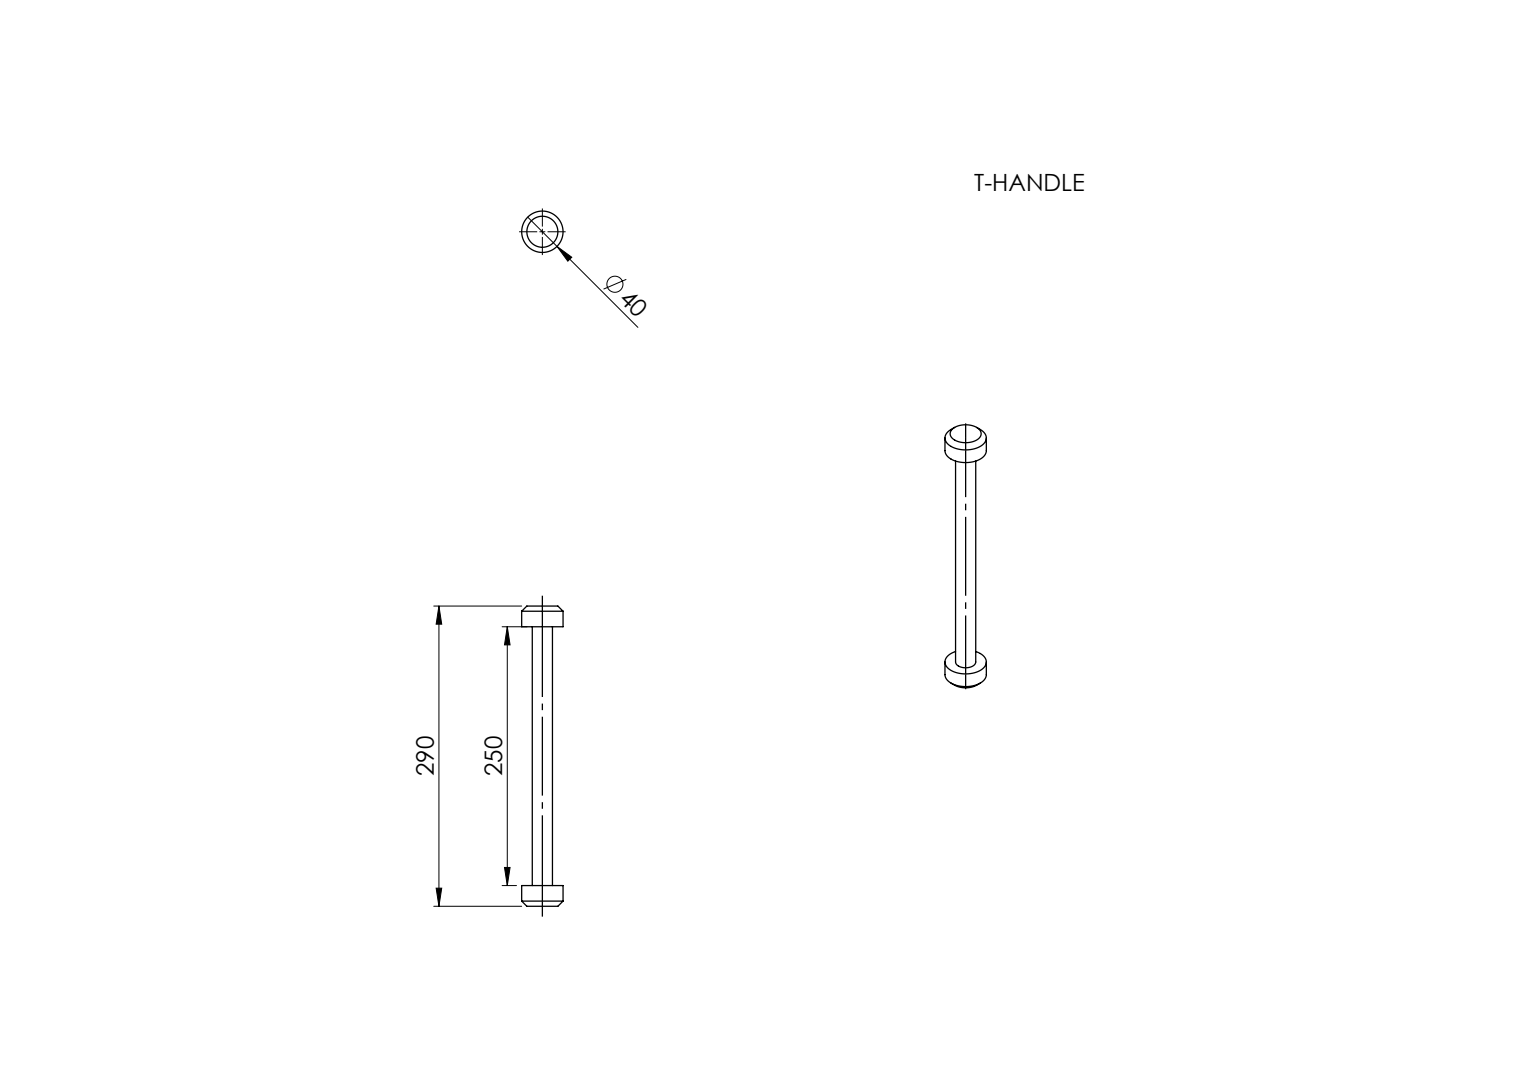
ISO-10303-21;
HEADER;
FILE_DESCRIPTION (('STEP AP203'),
    '1' );
FILE_NAME ('T-handle.step',
    '2026-09-28T05:57:06',
    ( '' ),
    ( '' ),
    'SwSTEP 2.0',
    'SolidWorks 2026',
    '' );
FILE_SCHEMA (( 'AUTOMOTIVE_DESIGN' ));
ENDSEC;

DATA;
#91=CARTESIAN_POINT ( 'NONE',  ( -1.040834085586084257E-14, -125.0000000000000000, 12.74999999999998934 ) ) ;
#177=LINE ( 'NONE', #29948, #5403 ) ;
#227=DIRECTION ( 'NONE',  ( 0.000000000000000000, -0.000000000000000000, 1.000000000000000000 ) ) ;
#268=ORIENTED_EDGE ( 'NONE', *, *, #28886, .F. ) ;
#419=VERTEX_POINT ( 'NONE', #17362 ) ;
#471=CARTESIAN_POINT ( 'NONE',  ( -1.040834085586084257E-14, -125.0000000000000000, 22.49999999999999289 ) ) ;
#473=ORIENTED_EDGE ( 'NONE', *, *, #25999, .F. ) ;
#566=CIRCLE ( 'NONE', #35714, 20.00000000000000000 ) ;
#851=MECHANICAL_CONTEXT ( 'NONE', #29772, 'mechanical' ) ;
#868=DIRECTION ( 'NONE',  ( 0.000000000000000000, 0.000000000000000000, -1.000000000000000000 ) ) ;
#1216=SHAPE_REPRESENTATION_RELATIONSHIP ( 'NONE' , 'NONE' ,  #40929, #17102 ) ;
#1231=DIRECTION ( 'NONE',  ( 0.000000000000000000, 0.000000000000000000, -1.000000000000000000 ) ) ;
#1234=CARTESIAN_POINT ( 'NONE',  ( -1.040834085586084257E-14, 145.0000000000000000, 22.49999999999999289 ) ) ;
#1383=LINE ( 'NONE', #34405, #18302 ) ;
#1425=DIRECTION ( 'NONE',  ( 0.000000000000000000, -1.000000000000000000, 0.000000000000000000 ) ) ;
#1545=LINE ( 'NONE', #40155, #18016 ) ;
#1660=CYLINDRICAL_SURFACE ( 'NONE', #36972, 20.00000000000000000 ) ;
#1786=CIRCLE ( 'NONE', #33508, 15.00000000000001066 ) ;
#1810=DIRECTION ( 'NONE',  ( 0.000000000000000000, 1.000000000000000000, 0.000000000000000000 ) ) ;
#1815=AXIS2_PLACEMENT_3D ( 'NONE', #36846, #20441, #33626 ) ;
#2067=CARTESIAN_POINT ( 'NONE',  ( -1.040834085586084257E-14, 139.9999999999999716, 2.499999999999992006 ) ) ;
#2073=ORIENTED_EDGE ( 'NONE', *, *, #14435, .F. ) ;
#2491=CARTESIAN_POINT ( 'NONE',  ( -1.040834085586084257E-14, 125.0000000000000000, 22.49999999999999289 ) ) ;
#3116=ORIENTED_EDGE ( 'NONE', *, *, #37024, .F. ) ;
#3335=VERTEX_POINT ( 'NONE', #22972 ) ;
#3448=EDGE_CURVE ( 'NONE', #21453, #419, #12086, .T. ) ;
#3451=CARTESIAN_POINT ( 'NONE',  ( -1.040834085586084257E-14, -145.0000000000000000, 22.49999999999999289 ) ) ;
#3477=DIRECTION ( 'NONE',  ( 0.000000000000000000, 0.000000000000000000, 1.000000000000000000 ) ) ;
#3738=LINE ( 'NONE', #6752, #8951 ) ;
#3889=CARTESIAN_POINT ( 'NONE',  ( -1.040834085586084257E-14, 145.0000000000000000, 22.49999999999999289 ) ) ;
#4161=ADVANCED_FACE ( 'NONE', ( #12961 ), #39308, .T. ) ;
#4188=DIRECTION ( 'NONE',  ( 0.000000000000000000, 1.000000000000000000, 0.000000000000000000 ) ) ;
#4342=VERTEX_POINT ( 'NONE', #5413 ) ;
#4391=FACE_OUTER_BOUND ( 'NONE', #42616, .T. ) ;
#4436=DIRECTION ( 'NONE',  ( 0.000000000000000000, 0.000000000000000000, 1.000000000000000000 ) ) ;
#4456=CYLINDRICAL_SURFACE ( 'NONE', #14879, 9.750000000000003553 ) ;
#4630=ORIENTED_EDGE ( 'NONE', *, *, #41333, .T. ) ;
#4816=EDGE_CURVE ( 'NONE', #28591, #27752, #8695, .T. ) ;
#4825=DIRECTION ( 'NONE',  ( -0.000000000000000000, -1.000000000000000000, -0.000000000000000000 ) ) ;
#4991=VECTOR ( 'NONE', #5574, 1000.000000000000000 ) ;
#5039=FACE_BOUND ( 'NONE', #22654, .T. ) ;
#5282=DIRECTION ( 'NONE',  ( 0.000000000000000000, 0.000000000000000000, 1.000000000000000000 ) ) ;
#5300=ORIENTED_EDGE ( 'NONE', *, *, #5846, .F. ) ;
#5341=ORIENTED_EDGE ( 'NONE', *, *, #32265, .F. ) ;
#5403=VECTOR ( 'NONE', #16964, 1000.000000000000000 ) ;
#5412=ADVANCED_FACE ( 'NONE', ( #20047 ), #40111, .T. ) ;
#5413=CARTESIAN_POINT ( 'NONE',  ( -1.040834085586084257E-14, -139.9999999999999716, 42.49999999999999289 ) ) ;
#5414=ADVANCED_FACE ( 'NONE', ( #13349, #26540 ), #39689, .F. ) ;
#5462=DIRECTION ( 'NONE',  ( 0.000000000000000000, 1.000000000000000000, 0.000000000000000000 ) ) ;
#5541=LINE ( 'NONE', #42409, #29579 ) ;
#5574=DIRECTION ( 'NONE',  ( -0.000000000000000000, 1.000000000000000000, -0.000000000000000000 ) ) ;
#5796=CARTESIAN_POINT ( 'NONE',  ( -1.040834085586084257E-14, 125.0000000000000000, 2.499999999999992006 ) ) ;
#5832=ORIENTED_EDGE ( 'NONE', *, *, #9357, .F. ) ;
#5846=EDGE_CURVE ( 'NONE', #39187, #5967, #12909, .T. ) ;
#5878=DIRECTION ( 'NONE',  ( 0.000000000000000000, 0.000000000000000000, -1.000000000000000000 ) ) ;
#5967=VERTEX_POINT ( 'NONE', #5796 ) ;
#6194=ORIENTED_EDGE ( 'NONE', *, *, #33703, .F. ) ;
#6272=DIRECTION ( 'NONE',  ( 0.000000000000000000, 0.000000000000000000, 1.000000000000000000 ) ) ;
#6295=AXIS2_PLACEMENT_3D ( 'NONE', #39092, #35241, #5878 ) ;
#6375=CARTESIAN_POINT ( 'NONE',  ( -8.571370657139810611E-15, -145.0000000000000000, 7.499999999999982236 ) ) ;
#6679=CARTESIAN_POINT ( 'NONE',  ( -8.265208957352971163E-15, -145.0000000000000000, 7.499999999999980460 ) ) ;
#6725=ORIENTED_EDGE ( 'NONE', *, *, #29092, .T. ) ;
#6752=CARTESIAN_POINT ( 'NONE',  ( -1.040834085586084257E-14, 125.0000000000000000, 12.74999999999998934 ) ) ;
#7066=CIRCLE ( 'NONE', #22933, 9.750000000000001776 ) ;
#7127=DIRECTION ( 'NONE',  ( -0.000000000000000000, -1.000000000000000000, -0.000000000000000000 ) ) ;
#7140=ORIENTED_EDGE ( 'NONE', *, *, #9357, .T. ) ;
#7254=FACE_OUTER_BOUND ( 'NONE', #12116, .T. ) ;
#7325=EDGE_CURVE ( 'NONE', #27752, #38572, #177, .T. ) ;
#7410=ORIENTED_EDGE ( 'NONE', *, *, #14435, .T. ) ;
#7450=AXIS2_PLACEMENT_3D ( 'NONE', #42023, #38585, #15478 ) ;
#7546=AXIS2_PLACEMENT_3D ( 'NONE', #35033, #5462, #15361 ) ;
#7648=DIRECTION ( 'NONE',  ( 0.000000000000000000, 0.000000000000000000, 1.000000000000000000 ) ) ;
#7735=AXIS2_PLACEMENT_3D ( 'NONE', #11600, #8398, #21548 ) ;
#7896=FACE_OUTER_BOUND ( 'NONE', #37238, .T. ) ;
#7974=FACE_OUTER_BOUND ( 'NONE', #12536, .T. ) ;
#8050=PRODUCT_DEFINITION_SHAPE ( 'NONE', 'NONE',  #24384 ) ;
#8094=ORIENTED_EDGE ( 'NONE', *, *, #32906, .F. ) ;
#8295=AXIS2_PLACEMENT_3D ( 'NONE', #20404, #1425, #41539 ) ;
#8353=FACE_OUTER_BOUND ( 'NONE', #19291, .T. ) ;
#8398=DIRECTION ( 'NONE',  ( 0.000000000000000000, -1.000000000000000000, 0.000000000000000000 ) ) ;
#8428=CYLINDRICAL_SURFACE ( 'NONE', #13259, 20.00000000000000355 ) ;
#8695=CIRCLE ( 'NONE', #1815, 14.99999999999998579 ) ;
#8706=ORIENTED_EDGE ( 'NONE', *, *, #5846, .T. ) ;
#8746=ORIENTED_EDGE ( 'NONE', *, *, #40574, .T. ) ;
#8807=ORIENTED_EDGE ( 'NONE', *, *, #31113, .T. ) ;
#8909=CARTESIAN_POINT ( 'NONE',  ( -7.959047257566134870E-15, 125.0000000000000000, 42.49999999999999289 ) ) ;
#8951=VECTOR ( 'NONE', #16868, 1000.000000000000000 ) ;
#9151=ORIENTED_EDGE ( 'NONE', *, *, #29092, .F. ) ;
#9230=CARTESIAN_POINT ( 'NONE',  ( -1.040834085586084257E-14, -139.9999999999999716, 22.49999999999999289 ) ) ;
#9234=DIRECTION ( 'NONE',  ( 0.000000000000000000, 0.000000000000000000, 1.000000000000000000 ) ) ;
#9270=ORIENTED_EDGE ( 'NONE', *, *, #18258, .F. ) ;
#9357=EDGE_CURVE ( 'NONE', #37654, #25583, #11643, .T. ) ;
#9744=CARTESIAN_POINT ( 'NONE',  ( -1.040834085586084257E-14, 145.0000000000000000, 22.49999999999999289 ) ) ;
#9794=CIRCLE ( 'NONE', #20826, 20.00000000000000355 ) ;
#10211=DIRECTION ( 'NONE',  ( 0.000000000000000000, 0.000000000000000000, -1.000000000000000000 ) ) ;
#10419=ORIENTED_EDGE ( 'NONE', *, *, #28886, .T. ) ;
#10429=UNCERTAINTY_MEASURE_WITH_UNIT (LENGTH_MEASURE( 1.000000000000000082E-05 ), #23882, 'distance_accuracy_value', 'NONE');
#10757=PRODUCT ( 'T-handle', 'T-handle', '', ( #851 ) ) ;
#10900=EDGE_CURVE ( 'NONE', #37654, #25373, #3738, .T. ) ;
#11112=DIRECTION ( 'NONE',  ( 0.000000000000000000, 0.000000000000000000, 1.000000000000000000 ) ) ;
#11370=ORIENTED_EDGE ( 'NONE', *, *, #37024, .T. ) ;
#11421=ORIENTED_EDGE ( 'NONE', *, *, #18258, .T. ) ;
#11600=CARTESIAN_POINT ( 'NONE',  ( -1.040834085586084257E-14, -145.0000000000000000, 22.49999999999999289 ) ) ;
#11643=CIRCLE ( 'NONE', #23396, 9.750000000000001776 ) ;
#12039=DIRECTION ( 'NONE',  ( 0.000000000000000000, 1.000000000000000000, 0.000000000000000000 ) ) ;
#12086=CIRCLE ( 'NONE', #29349, 15.00000000000001066 ) ;
#12116=EDGE_LOOP ( 'NONE', ( #15883, #7410, #35250, #37009 ) ) ;
#12183=EDGE_LOOP ( 'NONE', ( #16198, #17481, #11421, #28012 ) ) ;
#12520=DIRECTION ( 'NONE',  ( 0.000000000000000000, 0.000000000000000000, 1.000000000000000000 ) ) ;
#12536=EDGE_LOOP ( 'NONE', ( #2073, #42065, #22291, #32171 ) ) ;
#12645=CARTESIAN_POINT ( 'NONE',  ( -1.040834085586084257E-14, -145.0000000000000000, 42.49999999999999289 ) ) ;
#12873=CYLINDRICAL_SURFACE ( 'NONE', #7450, 9.750000000000003553 ) ;
#12909=CIRCLE ( 'NONE', #19152, 20.00000000000000355 ) ;
#12961=FACE_OUTER_BOUND ( 'NONE', #15238, .T. ) ;
#13031=LINE ( 'NONE', #6375, #28845 ) ;
#13034=AXIS2_PLACEMENT_3D ( 'NONE', #24309, #31209, #4436 ) ;
#13165=ORIENTED_EDGE ( 'NONE', *, *, #32906, .T. ) ;
#13259=AXIS2_PLACEMENT_3D ( 'NONE', #30871, #21581, #20715 ) ;
#13286=ORIENTED_EDGE ( 'NONE', *, *, #35143, .F. ) ;
#13349=FACE_BOUND ( 'NONE', #14661, .T. ) ;
#13398=EDGE_CURVE ( 'NONE', #27752, #28591, #24497, .T. ) ;
#13583=VERTEX_POINT ( 'NONE', #14542 ) ;
#13757=ADVANCED_FACE ( 'NONE', ( #5039, #4391 ), #18184, .F. ) ;
#13859=CIRCLE ( 'NONE', #6295, 20.00000000000000000 ) ;
#14121=( NAMED_UNIT ( * ) PLANE_ANGLE_UNIT ( ) SI_UNIT ( $, .RADIAN. ) );
#14435=EDGE_CURVE ( 'NONE', #28591, #34451, #1545, .T. ) ;
#14505=DIRECTION ( 'NONE',  ( 0.000000000000000000, -0.000000000000000000, 1.000000000000000000 ) ) ;
#14542=CARTESIAN_POINT ( 'NONE',  ( -9.214310226692173294E-15, -125.0000000000000000, 32.24999999999999289 ) ) ;
#14620=ORIENTED_EDGE ( 'NONE', *, *, #16955, .T. ) ;
#14661=EDGE_LOOP ( 'NONE', ( #6194, #9270 ) ) ;
#14780=ORIENTED_EDGE ( 'NONE', *, *, #27800, .F. ) ;
#14792=DIRECTION ( 'NONE',  ( -0.000000000000000000, -1.000000000000000000, -0.000000000000000000 ) ) ;
#14879=AXIS2_PLACEMENT_3D ( 'NONE', #21281, #30796, #1231 ) ;
#15101=DIRECTION ( 'NONE',  ( 0.000000000000000000, -1.000000000000000000, 0.000000000000000000 ) ) ;
#15238=EDGE_LOOP ( 'NONE', ( #15424, #36816, #11370, #14620 ) ) ;
#15361=DIRECTION ( 'NONE',  ( 0.000000000000000000, 0.000000000000000000, -1.000000000000000000 ) ) ;
#15424=ORIENTED_EDGE ( 'NONE', *, *, #19650, .F. ) ;
#15442=ORIENTED_EDGE ( 'NONE', *, *, #39183, .F. ) ;
#15478=DIRECTION ( 'NONE',  ( 0.000000000000000000, 0.000000000000000000, -1.000000000000000000 ) ) ;
#15625=ORIENTED_EDGE ( 'NONE', *, *, #31113, .F. ) ;
#15877=DIRECTION ( 'NONE',  ( 0.000000000000000000, -1.000000000000000000, 0.000000000000000000 ) ) ;
#15883=ORIENTED_EDGE ( 'NONE', *, *, #4816, .F. ) ;
#16198=ORIENTED_EDGE ( 'NONE', *, *, #40574, .F. ) ;
#16519=CIRCLE ( 'NONE', #30358, 9.750000000000001776 ) ;
#16610=AXIS2_PLACEMENT_3D ( 'NONE', #24461, #17732, #25103 ) ;
#16868=DIRECTION ( 'NONE',  ( -0.000000000000000000, -1.000000000000000000, -0.000000000000000000 ) ) ;
#16900=AXIS2_PLACEMENT_3D ( 'NONE', #9744, #22925, #17266 ) ;
#16955=EDGE_CURVE ( 'NONE', #5967, #39187, #9794, .T. ) ;
#16964=DIRECTION ( 'NONE',  ( 0.000000000000000000, -0.7071067811865487940, -0.7071067811865463515 ) ) ;
#17102=ADVANCED_BREP_SHAPE_REPRESENTATION ( '', ( #29300, #39998 ), #28294 ) ;
#17266=DIRECTION ( 'NONE',  ( 0.000000000000000000, 0.000000000000000000, -1.000000000000000000 ) ) ;
#17333=CARTESIAN_POINT ( 'NONE',  ( -1.040834085586084257E-14, -145.0000000000000000, 22.49999999999999289 ) ) ;
#17362=CARTESIAN_POINT ( 'NONE',  ( -1.040834085586084257E-14, -145.0000000000000000, 37.50000000000000711 ) ) ;
#17481=ORIENTED_EDGE ( 'NONE', *, *, #35143, .T. ) ;
#17732=DIRECTION ( 'NONE',  ( 0.000000000000000000, -1.000000000000000000, 0.000000000000000000 ) ) ;
#17992=DIRECTION ( 'NONE',  ( 0.000000000000000000, 0.000000000000000000, 1.000000000000000000 ) ) ;
#18016=VECTOR ( 'NONE', #30678, 1000.000000000000000 ) ;
#18184=PLANE ( 'NONE',  #29981 ) ;
#18258=EDGE_CURVE ( 'NONE', #13583, #25373, #7066, .T. ) ;
#18302=VECTOR ( 'NONE', #4825, 1000.000000000000000 ) ;
#18510=CONICAL_SURFACE ( 'NONE', #23327, 15.00000000000001421, 0.7853981633974469467 ) ;
#18565=ADVANCED_FACE ( 'NONE', ( #37984 ), #8428, .T. ) ;
#18586=CARTESIAN_POINT ( 'NONE',  ( -1.040834085586084257E-14, 125.0000000000000000, 22.49999999999999289 ) ) ;
#18658=DIRECTION ( 'NONE',  ( 0.000000000000000000, 1.000000000000000000, 0.000000000000000000 ) ) ;
#18945=FACE_OUTER_BOUND ( 'NONE', #33907, .T. ) ;
#19152=AXIS2_PLACEMENT_3D ( 'NONE', #32135, #12039, #9234 ) ;
#19291=EDGE_LOOP ( 'NONE', ( #4630, #39311, #8706, #3116 ) ) ;
#19323=EDGE_LOOP ( 'NONE', ( #8807, #6725, #10419, #14780 ) ) ;
#19345=CARTESIAN_POINT ( 'NONE',  ( -1.040834085586084257E-14, 145.0000000000000000, 7.500000000000003553 ) ) ;
#19362=CARTESIAN_POINT ( 'NONE',  ( -7.959047257566134870E-15, -145.0000000000000000, 2.499999999999992006 ) ) ;
#19418=DIRECTION ( 'NONE',  ( 0.000000000000000000, 1.000000000000000000, 0.000000000000000000 ) ) ;
#19650=EDGE_CURVE ( 'NONE', #34451, #39187, #1383, .T. ) ;
#19715=CARTESIAN_POINT ( 'NONE',  ( -1.040834085586084257E-14, -145.0000000000000000, 22.49999999999999289 ) ) ;
#19834=CARTESIAN_POINT ( 'NONE',  ( -1.040834085586084257E-14, 145.0000000000000000, 22.49999999999999289 ) ) ;
#19857=AXIS2_PLACEMENT_3D ( 'NONE', #20371, #30962, #7648 ) ;
#19982=CONICAL_SURFACE ( 'NONE', #8295, 14.99999999999998579, 0.7853981633974466137 ) ;
#20047=FACE_OUTER_BOUND ( 'NONE', #35756, .T. ) ;
#20371=CARTESIAN_POINT ( 'NONE',  ( -1.040834085586084257E-14, -125.0000000000000000, 22.49999999999999289 ) ) ;
#20404=CARTESIAN_POINT ( 'NONE',  ( -1.040834085586084257E-14, 145.0000000000000000, 22.49999999999999289 ) ) ;
#20441=DIRECTION ( 'NONE',  ( 0.000000000000000000, 1.000000000000000000, 0.000000000000000000 ) ) ;
#20539=CARTESIAN_POINT ( 'NONE',  ( -7.959047257566134870E-15, 139.9999999999999716, 42.49999999999999289 ) ) ;
#20576=DIRECTION ( 'NONE',  ( 0.000000000000000000, 0.000000000000000000, 1.000000000000000000 ) ) ;
#20624=CIRCLE ( 'NONE', #7546, 20.00000000000000000 ) ;
#20715=DIRECTION ( 'NONE',  ( 0.000000000000000000, 0.000000000000000000, 1.000000000000000000 ) ) ;
#20793=FACE_OUTER_BOUND ( 'NONE', #25894, .T. ) ;
#20826=AXIS2_PLACEMENT_3D ( 'NONE', #37652, #21456, #17992 ) ;
#20837=ORIENTED_EDGE ( 'NONE', *, *, #33703, .T. ) ;
#20943=EDGE_CURVE ( 'NONE', #419, #21453, #1786, .T. ) ;
#21048=( NAMED_UNIT ( * ) SI_UNIT ( $, .STERADIAN. ) SOLID_ANGLE_UNIT ( ) );
#21110=PLANE ( 'NONE',  #7735 ) ;
#21281=CARTESIAN_POINT ( 'NONE',  ( -1.040834085586084257E-14, 125.0000000000000000, 22.49999999999999289 ) ) ;
#21453=VERTEX_POINT ( 'NONE', #6679 ) ;
#21456=DIRECTION ( 'NONE',  ( 0.000000000000000000, 1.000000000000000000, 0.000000000000000000 ) ) ;
#21498=CONICAL_SURFACE ( 'NONE', #40096, 15.00000000000001421, 0.7853981633974469467 ) ;
#21548=DIRECTION ( 'NONE',  ( 0.000000000000000000, -0.000000000000000000, -1.000000000000000000 ) ) ;
#21581=DIRECTION ( 'NONE',  ( -0.000000000000000000, 1.000000000000000000, -0.000000000000000000 ) ) ;
#21733=CONICAL_SURFACE ( 'NONE', #36204, 14.99999999999998579, 0.7853981633974466137 ) ;
#22009=ADVANCED_FACE ( 'NONE', ( #27338 ), #4456, .T. ) ;
#22291=ORIENTED_EDGE ( 'NONE', *, *, #7325, .T. ) ;
#22512=ADVANCED_FACE ( 'NONE', ( #8353 ), #1660, .T. ) ;
#22513=CARTESIAN_POINT ( 'NONE',  ( -1.040834085586084257E-14, -145.0000000000000000, 37.50000000000000711 ) ) ;
#22594=LINE ( 'NONE', #12645, #28388 ) ;
#22608=DIRECTION ( 'NONE',  ( 0.000000000000000000, -1.000000000000000000, 0.000000000000000000 ) ) ;
#22654=EDGE_LOOP ( 'NONE', ( #7140, #8746 ) ) ;
#22925=DIRECTION ( 'NONE',  ( -0.000000000000000000, -1.000000000000000000, -0.000000000000000000 ) ) ;
#22933=AXIS2_PLACEMENT_3D ( 'NONE', #471, #26983, #3477 ) ;
#22972=CARTESIAN_POINT ( 'NONE',  ( -7.959047257566134870E-15, -125.0000000000000000, 2.499999999999992006 ) ) ;
#23303=CARTESIAN_POINT ( 'NONE',  ( -1.040834085586084257E-14, -125.0000000000000000, 22.49999999999999289 ) ) ;
#23327=AXIS2_PLACEMENT_3D ( 'NONE', #17333, #4188, #20576 ) ;
#23396=AXIS2_PLACEMENT_3D ( 'NONE', #18586, #28532, #12520 ) ;
#23614=ADVANCED_FACE ( 'NONE', ( #7974 ), #21733, .T. ) ;
#23882=( LENGTH_UNIT ( ) NAMED_UNIT ( * ) SI_UNIT ( .MILLI., .METRE. ) );
#24309=CARTESIAN_POINT ( 'NONE',  ( -1.040834085586084257E-14, -145.0000000000000000, 22.49999999999999289 ) ) ;
#24384=PRODUCT_DEFINITION ( 'UNKNOWN', '', #28392, #39072 ) ;
#24461=CARTESIAN_POINT ( 'NONE',  ( -1.040834085586084257E-14, 139.9999999999999716, 22.49999999999999289 ) ) ;
#24470=AXIS2_PLACEMENT_3D ( 'NONE', #31409, #34860, #5282 ) ;
#24497=CIRCLE ( 'NONE', #24470, 14.99999999999998579 ) ;
#24743=CARTESIAN_POINT ( 'NONE',  ( 0.000000000000000000, 0.000000000000000000, 0.000000000000000000 ) ) ;
#25103=DIRECTION ( 'NONE',  ( 0.000000000000000000, 0.000000000000000000, 1.000000000000000000 ) ) ;
#25167=ORIENTED_EDGE ( 'NONE', *, *, #4816, .T. ) ;
#25227=CARTESIAN_POINT ( 'NONE',  ( -1.040834085586084257E-14, -125.0000000000000000, 22.49999999999999289 ) ) ;
#25373=VERTEX_POINT ( 'NONE', #91 ) ;
#25583=VERTEX_POINT ( 'NONE', #27471 ) ;
#25843=EDGE_CURVE ( 'NONE', #34451, #38572, #34575, .T. ) ;
#25894=EDGE_LOOP ( 'NONE', ( #32902, #28883, #15625, #8094 ) ) ;
#25999=EDGE_CURVE ( 'NONE', #32995, #3335, #13859, .T. ) ;
#26540=FACE_OUTER_BOUND ( 'NONE', #32275, .T. ) ;
#26766=LINE ( 'NONE', #39919, #30255 ) ;
#26956=DIRECTION ( 'NONE',  ( 0.000000000000000000, 1.000000000000000000, 0.000000000000000000 ) ) ;
#26983=DIRECTION ( 'NONE',  ( 0.000000000000000000, 1.000000000000000000, 0.000000000000000000 ) ) ;
#26991=ADVANCED_FACE ( 'NONE', ( #29569 ), #21498, .T. ) ;
#27338=FACE_OUTER_BOUND ( 'NONE', #12183, .T. ) ;
#27471=CARTESIAN_POINT ( 'NONE',  ( -9.214310226692173294E-15, 125.0000000000000000, 32.24999999999999289 ) ) ;
#27752=VERTEX_POINT ( 'NONE', #19345 ) ;
#27800=EDGE_CURVE ( 'NONE', #4342, #32995, #22594, .T. ) ;
#27987=DIRECTION ( 'NONE',  ( 0.000000000000000000, 0.000000000000000000, -1.000000000000000000 ) ) ;
#28012=ORIENTED_EDGE ( 'NONE', *, *, #10900, .F. ) ;
#28294=( GEOMETRIC_REPRESENTATION_CONTEXT ( 3 ) GLOBAL_UNCERTAINTY_ASSIGNED_CONTEXT ( ( #10429 ) ) GLOBAL_UNIT_ASSIGNED_CONTEXT ( ( #23882, #14121, #21048 ) ) REPRESENTATION_CONTEXT ( 'NONE', 'WORKASPACE' ) );
#28388=VECTOR ( 'NONE', #38993, 1000.000000000000000 ) ;
#28392=PRODUCT_DEFINITION_FORMATION_WITH_SPECIFIED_SOURCE ( 'ANY', '', #10757, .NOT_KNOWN. ) ;
#28403=ORIENTED_EDGE ( 'NONE', *, *, #39183, .T. ) ;
#28532=DIRECTION ( 'NONE',  ( 0.000000000000000000, 1.000000000000000000, 0.000000000000000000 ) ) ;
#28591=VERTEX_POINT ( 'NONE', #40945 ) ;
#28677=DIRECTION ( 'NONE',  ( 0.000000000000000000, 0.000000000000000000, -1.000000000000000000 ) ) ;
#28755=ADVANCED_FACE ( 'NONE', ( #37952 ), #21110, .T. ) ;
#28790=LINE ( 'NONE', #22513, #34355 ) ;
#28845=VECTOR ( 'NONE', #39167, 1000.000000000000000 ) ;
#28883=ORIENTED_EDGE ( 'NONE', *, *, #32265, .T. ) ;
#28886=EDGE_CURVE ( 'NONE', #3335, #32995, #29793, .T. ) ;
#29092=EDGE_CURVE ( 'NONE', #32177, #3335, #42233, .T. ) ;
#29290=ORIENTED_EDGE ( 'NONE', *, *, #13398, .T. ) ;
#29300=MANIFOLD_SOLID_BREP ( 'Chamfer1', #41117 ) ;
#29349=AXIS2_PLACEMENT_3D ( 'NONE', #19715, #29873, #10211 ) ;
#29569=FACE_OUTER_BOUND ( 'NONE', #33567, .T. ) ;
#29579=VECTOR ( 'NONE', #36159, 1000.000000000000000 ) ;
#29772=APPLICATION_CONTEXT ( 'configuration controlled 3d designs of mechanical parts and assemblies' ) ;
#29793=CIRCLE ( 'NONE', #39423, 20.00000000000000000 ) ;
#29873=DIRECTION ( 'NONE',  ( 0.000000000000000000, -1.000000000000000000, 0.000000000000000000 ) ) ;
#29948=CARTESIAN_POINT ( 'NONE',  ( -1.040834085586084257E-14, 145.0000000000000000, 7.500000000000007105 ) ) ;
#29981=AXIS2_PLACEMENT_3D ( 'NONE', #31376, #1810, #14505 ) ;
#30058=CARTESIAN_POINT ( 'NONE',  ( -1.040834085586084257E-14, -125.0000000000000000, 42.49999999999999289 ) ) ;
#30255=VECTOR ( 'NONE', #7127, 1000.000000000000000 ) ;
#30358=AXIS2_PLACEMENT_3D ( 'NONE', #2491, #18658, #41742 ) ;
#30437=DIRECTION ( 'NONE',  ( 0.000000000000000000, -1.000000000000000000, 0.000000000000000000 ) ) ;
#30678=DIRECTION ( 'NONE',  ( 8.659560562354918067E-17, -0.7071067811865487940, 0.7071067811865463515 ) ) ;
#30796=DIRECTION ( 'NONE',  ( -0.000000000000000000, -1.000000000000000000, -0.000000000000000000 ) ) ;
#30871=CARTESIAN_POINT ( 'NONE',  ( -1.040834085586084257E-14, -145.0000000000000000, 22.49999999999999289 ) ) ;
#30933=ORIENTED_EDGE ( 'NONE', *, *, #20943, .F. ) ;
#30962=DIRECTION ( 'NONE',  ( 0.000000000000000000, 1.000000000000000000, 0.000000000000000000 ) ) ;
#31106=ORIENTED_EDGE ( 'NONE', *, *, #10900, .T. ) ;
#31113=EDGE_CURVE ( 'NONE', #4342, #32177, #566, .T. ) ;
#31209=DIRECTION ( 'NONE',  ( -0.000000000000000000, 1.000000000000000000, -0.000000000000000000 ) ) ;
#31262=ADVANCED_FACE ( 'NONE', ( #18945 ), #12873, .T. ) ;
#31376=CARTESIAN_POINT ( 'NONE',  ( -1.040834085586084257E-14, 125.0000000000000000, 22.49999999999999289 ) ) ;
#31386=DIRECTION ( 'NONE',  ( 0.000000000000000000, 0.7071067811865484609, 0.7071067811865465735 ) ) ;
#31409=CARTESIAN_POINT ( 'NONE',  ( -1.040834085586084257E-14, 145.0000000000000000, 22.49999999999999289 ) ) ;
#31544=CARTESIAN_POINT ( 'NONE',  ( -1.040834085586084257E-14, -145.0000000000000000, 22.49999999999999289 ) ) ;
#32135=CARTESIAN_POINT ( 'NONE',  ( -1.040834085586084257E-14, 125.0000000000000000, 22.49999999999999289 ) ) ;
#32171=ORIENTED_EDGE ( 'NONE', *, *, #25843, .F. ) ;
#32177=VERTEX_POINT ( 'NONE', #32499 ) ;
#32265=EDGE_CURVE ( 'NONE', #21453, #32177, #13031, .T. ) ;
#32275=EDGE_LOOP ( 'NONE', ( #473, #268 ) ) ;
#32499=CARTESIAN_POINT ( 'NONE',  ( -7.959047257566134870E-15, -139.9999999999999716, 2.499999999999992006 ) ) ;
#32505=ADVANCED_FACE ( 'NONE', ( #20793 ), #18510, .T. ) ;
#32902=ORIENTED_EDGE ( 'NONE', *, *, #3448, .F. ) ;
#32906=EDGE_CURVE ( 'NONE', #419, #4342, #28790, .T. ) ;
#32995=VERTEX_POINT ( 'NONE', #30058 ) ;
#33242=DIRECTION ( 'NONE',  ( 0.000000000000000000, -0.000000000000000000, -1.000000000000000000 ) ) ;
#33508=AXIS2_PLACEMENT_3D ( 'NONE', #31544, #15101, #40787 ) ;
#33544=EDGE_LOOP ( 'NONE', ( #40730, #40717 ) ) ;
#33567=EDGE_LOOP ( 'NONE', ( #5341, #30933, #13165, #15442 ) ) ;
#33626=DIRECTION ( 'NONE',  ( 0.000000000000000000, 0.000000000000000000, 1.000000000000000000 ) ) ;
#33703=EDGE_CURVE ( 'NONE', #25373, #13583, #35040, .T. ) ;
#33804=AXIS2_PLACEMENT_3D ( 'NONE', #42427, #15877, #38991 ) ;
#33907=EDGE_LOOP ( 'NONE', ( #13286, #5832, #31106, #20837 ) ) ;
#34355=VECTOR ( 'NONE', #31386, 1000.000000000000000 ) ;
#34405=CARTESIAN_POINT ( 'NONE',  ( -7.959047257566134870E-15, 145.0000000000000000, 42.49999999999999289 ) ) ;
#34451=VERTEX_POINT ( 'NONE', #20539 ) ;
#34575=CIRCLE ( 'NONE', #16610, 20.00000000000000355 ) ;
#34665=CARTESIAN_POINT ( 'NONE',  ( -1.040834085586084257E-14, 125.0000000000000000, 12.74999999999998934 ) ) ;
#34725=SHAPE_DEFINITION_REPRESENTATION ( #8050, #40929 ) ;
#34860=DIRECTION ( 'NONE',  ( 0.000000000000000000, 1.000000000000000000, 0.000000000000000000 ) ) ;
#35033=CARTESIAN_POINT ( 'NONE',  ( -1.040834085586084257E-14, -139.9999999999999716, 22.49999999999999289 ) ) ;
#35040=CIRCLE ( 'NONE', #19857, 9.750000000000001776 ) ;
#35143=EDGE_CURVE ( 'NONE', #25583, #13583, #26766, .T. ) ;
#35241=DIRECTION ( 'NONE',  ( 0.000000000000000000, -1.000000000000000000, 0.000000000000000000 ) ) ;
#35250=ORIENTED_EDGE ( 'NONE', *, *, #41333, .F. ) ;
#35714=AXIS2_PLACEMENT_3D ( 'NONE', #9230, #41603, #38377 ) ;
#35756=EDGE_LOOP ( 'NONE', ( #29290, #25167 ) ) ;
#36159=DIRECTION ( 'NONE',  ( -0.000000000000000000, -1.000000000000000000, -0.000000000000000000 ) ) ;
#36204=AXIS2_PLACEMENT_3D ( 'NONE', #3889, #30437, #868 ) ;
#36285=ORIENTED_EDGE ( 'NONE', *, *, #16955, .F. ) ;
#36816=ORIENTED_EDGE ( 'NONE', *, *, #25843, .T. ) ;
#36846=CARTESIAN_POINT ( 'NONE',  ( -1.040834085586084257E-14, 145.0000000000000000, 22.49999999999999289 ) ) ;
#36972=AXIS2_PLACEMENT_3D ( 'NONE', #1234, #14792, #27987 ) ;
#37009=ORIENTED_EDGE ( 'NONE', *, *, #7325, .F. ) ;
#37024=EDGE_CURVE ( 'NONE', #38572, #5967, #5541, .T. ) ;
#37238=EDGE_LOOP ( 'NONE', ( #9151, #28403, #40355, #42120 ) ) ;
#37629=AXIS2_PLACEMENT_3D ( 'NONE', #23303, #39269, #33242 ) ;
#37652=CARTESIAN_POINT ( 'NONE',  ( -1.040834085586084257E-14, 125.0000000000000000, 22.49999999999999289 ) ) ;
#37654=VERTEX_POINT ( 'NONE', #34665 ) ;
#37889=DIRECTION ( 'NONE',  ( 1.000000000000000000, 0.000000000000000000, 0.000000000000000000 ) ) ;
#37952=FACE_OUTER_BOUND ( 'NONE', #33544, .T. ) ;
#37984=FACE_OUTER_BOUND ( 'NONE', #19323, .T. ) ;
#38345=ADVANCED_FACE ( 'NONE', ( #7896 ), #41311, .T. ) ;
#38377=DIRECTION ( 'NONE',  ( 0.000000000000000000, 0.000000000000000000, -1.000000000000000000 ) ) ;
#38572=VERTEX_POINT ( 'NONE', #2067 ) ;
#38585=DIRECTION ( 'NONE',  ( -0.000000000000000000, -1.000000000000000000, -0.000000000000000000 ) ) ;
#38635=CIRCLE ( 'NONE', #33804, 20.00000000000000355 ) ;
#38991=DIRECTION ( 'NONE',  ( 0.000000000000000000, 0.000000000000000000, 1.000000000000000000 ) ) ;
#38993=DIRECTION ( 'NONE',  ( -0.000000000000000000, 1.000000000000000000, -0.000000000000000000 ) ) ;
#39072=DESIGN_CONTEXT ( 'detailed design', #42159, 'design' ) ;
#39092=CARTESIAN_POINT ( 'NONE',  ( -1.040834085586084257E-14, -125.0000000000000000, 22.49999999999999289 ) ) ;
#39167=DIRECTION ( 'NONE',  ( 8.659560562354921765E-17, 0.7071067811865484609, -0.7071067811865465735 ) ) ;
#39183=EDGE_CURVE ( 'NONE', #32177, #4342, #20624, .T. ) ;
#39187=VERTEX_POINT ( 'NONE', #8909 ) ;
#39269=DIRECTION ( 'NONE',  ( 0.000000000000000000, -1.000000000000000000, 0.000000000000000000 ) ) ;
#39308=CYLINDRICAL_SURFACE ( 'NONE', #16900, 20.00000000000000000 ) ;
#39311=ORIENTED_EDGE ( 'NONE', *, *, #19650, .T. ) ;
#39423=AXIS2_PLACEMENT_3D ( 'NONE', #25227, #22608, #28677 ) ;
#39689=PLANE ( 'NONE',  #37629 ) ;
#39919=CARTESIAN_POINT ( 'NONE',  ( -9.214310226692173294E-15, 125.0000000000000000, 32.24999999999999289 ) ) ;
#39998=AXIS2_PLACEMENT_3D ( 'NONE', #24743, #11112, #37889 ) ;
#40096=AXIS2_PLACEMENT_3D ( 'NONE', #3451, #19418, #6272 ) ;
#40111=PLANE ( 'NONE',  #41051 ) ;
#40155=CARTESIAN_POINT ( 'NONE',  ( -8.571370657139813766E-15, 145.0000000000000000, 37.49999999999997868 ) ) ;
#40305=ADVANCED_FACE ( 'NONE', ( #7254 ), #19982, .T. ) ;
#40355=ORIENTED_EDGE ( 'NONE', *, *, #27800, .T. ) ;
#40574=EDGE_CURVE ( 'NONE', #25583, #37654, #16519, .T. ) ;
#40717=ORIENTED_EDGE ( 'NONE', *, *, #3448, .T. ) ;
#40730=ORIENTED_EDGE ( 'NONE', *, *, #20943, .T. ) ;
#40787=DIRECTION ( 'NONE',  ( 0.000000000000000000, 0.000000000000000000, -1.000000000000000000 ) ) ;
#40929=SHAPE_REPRESENTATION ( 'T-handle', ( #39998 ), #28294 ) ;
#40945=CARTESIAN_POINT ( 'NONE',  ( -8.265208957352974318E-15, 145.0000000000000000, 37.49999999999997868 ) ) ;
#41051=AXIS2_PLACEMENT_3D ( 'NONE', #19834, #26956, #227 ) ;
#41117=CLOSED_SHELL ( 'NONE', ( #32505, #40305, #22512, #18565, #22009, #31262, #38345, #28755, #5414, #4161, #5412, #13757, #23614, #26991 ) ) ;
#41311=CYLINDRICAL_SURFACE ( 'NONE', #13034, 20.00000000000000355 ) ;
#41333=EDGE_CURVE ( 'NONE', #38572, #34451, #38635, .T. ) ;
#41539=DIRECTION ( 'NONE',  ( 0.000000000000000000, 0.000000000000000000, -1.000000000000000000 ) ) ;
#41603=DIRECTION ( 'NONE',  ( 0.000000000000000000, 1.000000000000000000, 0.000000000000000000 ) ) ;
#41742=DIRECTION ( 'NONE',  ( 0.000000000000000000, 0.000000000000000000, 1.000000000000000000 ) ) ;
#42023=CARTESIAN_POINT ( 'NONE',  ( -1.040834085586084257E-14, 125.0000000000000000, 22.49999999999999289 ) ) ;
#42065=ORIENTED_EDGE ( 'NONE', *, *, #13398, .F. ) ;
#42120=ORIENTED_EDGE ( 'NONE', *, *, #25999, .T. ) ;
#42159=APPLICATION_CONTEXT ( 'configuration controlled 3d designs of mechanical parts and assemblies' ) ;
#42233=LINE ( 'NONE', #19362, #4991 ) ;
#42409=CARTESIAN_POINT ( 'NONE',  ( -1.040834085586084257E-14, 145.0000000000000000, 2.499999999999992006 ) ) ;
#42427=CARTESIAN_POINT ( 'NONE',  ( -1.040834085586084257E-14, 139.9999999999999716, 22.49999999999999289 ) ) ;
#42616=EDGE_LOOP ( 'NONE', ( #36285, #5300 ) ) ;
#42718=COLOUR_RGB('Slate Gray', 0.40784314, 0.44705882, 0.49803922);
#42719=FILL_AREA_STYLE_COLOUR('',#42718);
#42720=FILL_AREA_STYLE('',(#42719));
#42721=SURFACE_STYLE_FILL_AREA(#42720);
#42722=SURFACE_SIDE_STYLE('',(#42721));
#42723=SURFACE_STYLE_USAGE(.BOTH.,#42722);
#42724=PRESENTATION_STYLE_ASSIGNMENT((#42723));
#42741=STYLED_ITEM('',(#42724),#29300);
#42742=MECHANICAL_DESIGN_GEOMETRIC_PRESENTATION_REPRESENTATION('',(#42741),#28294);
ENDSEC;
END-ISO-10303-21;
